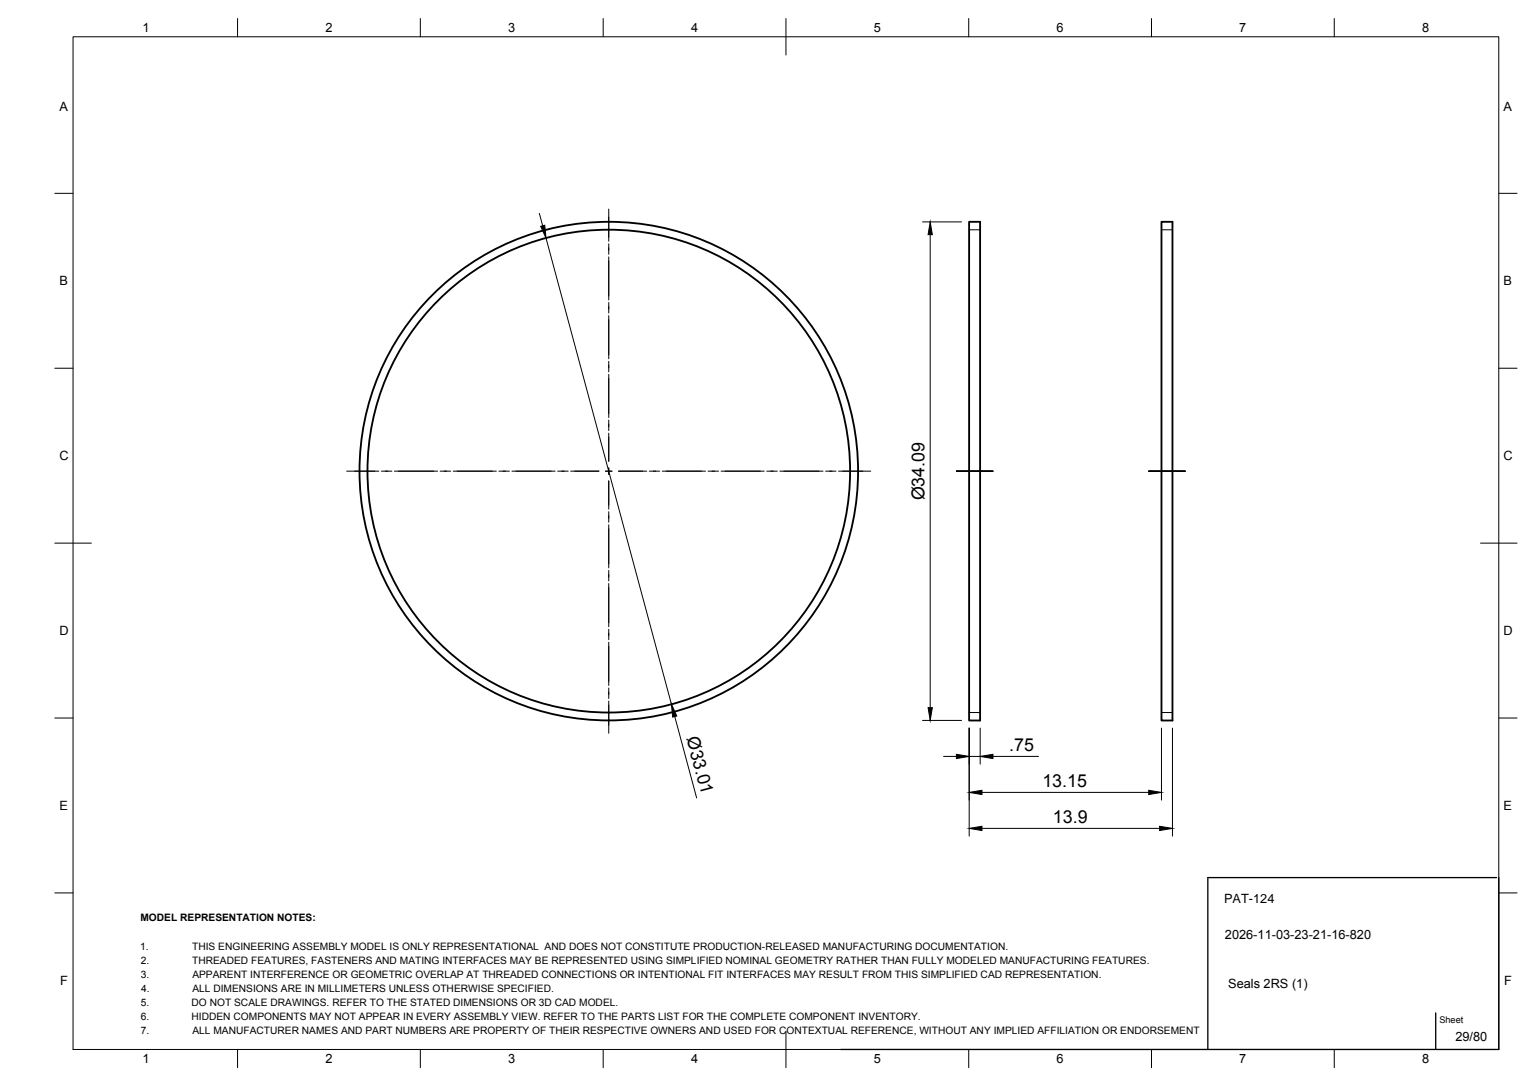
ISO-10303-21;
HEADER;
/* Generated by software containing ST-Developer
 * from STEP Tools, Inc. (www.steptools.com) 
 */

FILE_DESCRIPTION(
/* description */ ('XY cross-slide table'),
/* implementation_level */ '2;1');

FILE_NAME(
/* name */ 'Seals 2RS (1).step',
/* time_stamp */ '2026-10-28T03:22:46-07:00',
/* author */ (''),
/* organization */ (''),
/* preprocessor_version */ 'ST-DEVELOPER v20.2',
/* originating_system */ 'Autodesk Translation Framework v15.17.0.0',
/* authorisation */ '');

FILE_SCHEMA (('AUTOMOTIVE_DESIGN { 1 0 10303 214 3 1 1 }'));
ENDSEC;

DATA;
#10=MECHANICAL_DESIGN_GEOMETRIC_PRESENTATION_REPRESENTATION('',(#1704,#1705),#62984);
#1524=SHAPE_REPRESENTATION_RELATIONSHIP('SRR','None',#63374,#1607);
#1607=ADVANCED_BREP_SHAPE_REPRESENTATION('',(#1817,#1818),#62911);
#1704=STYLED_ITEM('',(#63912),#1817);
#1705=STYLED_ITEM('',(#63912),#1818);
#1817=MANIFOLD_SOLID_BREP('Body1',#22998);
#1818=MANIFOLD_SOLID_BREP('Body2',#22999);
#1997=FACE_BOUND('',#4532,.T.);
#1998=FACE_BOUND('',#4535,.T.);
#1999=FACE_BOUND('',#4538,.T.);
#2000=FACE_BOUND('',#4541,.T.);
#2410=PLANE('',#24526);
#2411=PLANE('',#24531);
#2412=PLANE('',#24534);
#2413=PLANE('',#24539);
#3107=FACE_OUTER_BOUND('',#4531,.T.);
#3108=FACE_OUTER_BOUND('',#4533,.T.);
#3109=FACE_OUTER_BOUND('',#4534,.T.);
#3110=FACE_OUTER_BOUND('',#4536,.T.);
#3111=FACE_OUTER_BOUND('',#4537,.T.);
#3112=FACE_OUTER_BOUND('',#4539,.T.);
#3113=FACE_OUTER_BOUND('',#4540,.T.);
#3114=FACE_OUTER_BOUND('',#4542,.T.);
#4531=EDGE_LOOP('',(#15940));
#4532=EDGE_LOOP('',(#15941));
#4533=EDGE_LOOP('',(#15942,#15943,#15944,#15945));
#4534=EDGE_LOOP('',(#15946));
#4535=EDGE_LOOP('',(#15947));
#4536=EDGE_LOOP('',(#15948,#15949,#15950,#15951));
#4537=EDGE_LOOP('',(#15952));
#4538=EDGE_LOOP('',(#15953));
#4539=EDGE_LOOP('',(#15954,#15955,#15956,#15957));
#4540=EDGE_LOOP('',(#15958));
#4541=EDGE_LOOP('',(#15959));
#4542=EDGE_LOOP('',(#15960,#15961,#15962,#15963));
#6135=LINE('',#34657,#7622);
#6136=LINE('',#34662,#7623);
#6137=LINE('',#34671,#7624);
#6138=LINE('',#34676,#7625);
#7622=VECTOR('',#27752,1.70469);
#7623=VECTOR('',#27759,1.65031);
#7624=VECTOR('',#27770,1.70469);
#7625=VECTOR('',#27777,1.65031);
#9137=CIRCLE('',#24527,1.70469);
#9138=CIRCLE('',#24528,1.65031);
#9139=CIRCLE('',#24530,1.70469);
#9140=CIRCLE('',#24532,1.65031);
#9141=CIRCLE('',#24535,1.70469);
#9142=CIRCLE('',#24536,1.65031);
#9143=CIRCLE('',#24538,1.70469);
#9144=CIRCLE('',#24540,1.65031);
#10133=VERTEX_POINT('',#34650);
#10134=VERTEX_POINT('',#34652);
#10135=VERTEX_POINT('',#34655);
#10136=VERTEX_POINT('',#34659);
#10137=VERTEX_POINT('',#34664);
#10138=VERTEX_POINT('',#34666);
#10139=VERTEX_POINT('',#34669);
#10140=VERTEX_POINT('',#34673);
#12354=EDGE_CURVE('',#10133,#10133,#9137,.T.);
#12355=EDGE_CURVE('',#10134,#10134,#9138,.T.);
#12356=EDGE_CURVE('',#10135,#10135,#9139,.T.);
#12357=EDGE_CURVE('',#10135,#10133,#6135,.T.);
#12358=EDGE_CURVE('',#10136,#10136,#9140,.T.);
#12359=EDGE_CURVE('',#10136,#10134,#6136,.T.);
#12360=EDGE_CURVE('',#10137,#10137,#9141,.T.);
#12361=EDGE_CURVE('',#10138,#10138,#9142,.T.);
#12362=EDGE_CURVE('',#10139,#10139,#9143,.T.);
#12363=EDGE_CURVE('',#10139,#10137,#6137,.T.);
#12364=EDGE_CURVE('',#10140,#10140,#9144,.T.);
#12365=EDGE_CURVE('',#10140,#10138,#6138,.T.);
#15940=ORIENTED_EDGE('',*,*,#12354,.F.);
#15941=ORIENTED_EDGE('',*,*,#12355,.T.);
#15942=ORIENTED_EDGE('',*,*,#12356,.F.);
#15943=ORIENTED_EDGE('',*,*,#12357,.T.);
#15944=ORIENTED_EDGE('',*,*,#12354,.T.);
#15945=ORIENTED_EDGE('',*,*,#12357,.F.);
#15946=ORIENTED_EDGE('',*,*,#12356,.T.);
#15947=ORIENTED_EDGE('',*,*,#12358,.F.);
#15948=ORIENTED_EDGE('',*,*,#12358,.T.);
#15949=ORIENTED_EDGE('',*,*,#12359,.T.);
#15950=ORIENTED_EDGE('',*,*,#12355,.F.);
#15951=ORIENTED_EDGE('',*,*,#12359,.F.);
#15952=ORIENTED_EDGE('',*,*,#12360,.F.);
#15953=ORIENTED_EDGE('',*,*,#12361,.T.);
#15954=ORIENTED_EDGE('',*,*,#12362,.F.);
#15955=ORIENTED_EDGE('',*,*,#12363,.T.);
#15956=ORIENTED_EDGE('',*,*,#12360,.T.);
#15957=ORIENTED_EDGE('',*,*,#12363,.F.);
#15958=ORIENTED_EDGE('',*,*,#12362,.T.);
#15959=ORIENTED_EDGE('',*,*,#12364,.F.);
#15960=ORIENTED_EDGE('',*,*,#12364,.T.);
#15961=ORIENTED_EDGE('',*,*,#12365,.T.);
#15962=ORIENTED_EDGE('',*,*,#12361,.F.);
#15963=ORIENTED_EDGE('',*,*,#12365,.F.);
#21122=CYLINDRICAL_SURFACE('',#24529,1.70469);
#21123=CYLINDRICAL_SURFACE('',#24533,1.65031);
#21124=CYLINDRICAL_SURFACE('',#24537,1.70469);
#21125=CYLINDRICAL_SURFACE('',#24541,1.65031);
#21888=ADVANCED_FACE('',(#3107,#1997),#2410,.T.);
#21889=ADVANCED_FACE('',(#3108),#21122,.T.);
#21890=ADVANCED_FACE('',(#3109,#1998),#2411,.T.);
#21891=ADVANCED_FACE('',(#3110),#21123,.F.);
#21892=ADVANCED_FACE('',(#3111,#1999),#2412,.T.);
#21893=ADVANCED_FACE('',(#3112),#21124,.T.);
#21894=ADVANCED_FACE('',(#3113,#2000),#2413,.T.);
#21895=ADVANCED_FACE('',(#3114),#21125,.F.);
#22998=CLOSED_SHELL('',(#21888,#21889,#21890,#21891));
#22999=CLOSED_SHELL('',(#21892,#21893,#21894,#21895));
#24525=AXIS2_PLACEMENT_3D('',#34648,#27740,#27741);
#24526=AXIS2_PLACEMENT_3D('',#34649,#27742,#27743);
#24527=AXIS2_PLACEMENT_3D('',#34651,#27744,#27745);
#24528=AXIS2_PLACEMENT_3D('',#34653,#27746,#27747);
#24529=AXIS2_PLACEMENT_3D('',#34654,#27748,#27749);
#24530=AXIS2_PLACEMENT_3D('',#34656,#27750,#27751);
#24531=AXIS2_PLACEMENT_3D('',#34658,#27753,#27754);
#24532=AXIS2_PLACEMENT_3D('',#34660,#27755,#27756);
#24533=AXIS2_PLACEMENT_3D('',#34661,#27757,#27758);
#24534=AXIS2_PLACEMENT_3D('',#34663,#27760,#27761);
#24535=AXIS2_PLACEMENT_3D('',#34665,#27762,#27763);
#24536=AXIS2_PLACEMENT_3D('',#34667,#27764,#27765);
#24537=AXIS2_PLACEMENT_3D('',#34668,#27766,#27767);
#24538=AXIS2_PLACEMENT_3D('',#34670,#27768,#27769);
#24539=AXIS2_PLACEMENT_3D('',#34672,#27771,#27772);
#24540=AXIS2_PLACEMENT_3D('',#34674,#27773,#27774);
#24541=AXIS2_PLACEMENT_3D('',#34675,#27775,#27776);
#27740=DIRECTION('axis',(0.,0.,1.));
#27741=DIRECTION('refdir',(1.,0.,0.));
#27742=DIRECTION('center_axis',(0.,1.,0.));
#27743=DIRECTION('ref_axis',(0.,0.,1.));
#27744=DIRECTION('center_axis',(0.,-1.,0.));
#27745=DIRECTION('ref_axis',(1.,0.,0.));
#27746=DIRECTION('center_axis',(0.,-1.,0.));
#27747=DIRECTION('ref_axis',(1.,0.,0.));
#27748=DIRECTION('center_axis',(0.,-1.,0.));
#27749=DIRECTION('ref_axis',(1.,0.,0.));
#27750=DIRECTION('center_axis',(0.,-1.,0.));
#27751=DIRECTION('ref_axis',(1.,0.,0.));
#27752=DIRECTION('',(0.,1.,0.));
#27753=DIRECTION('center_axis',(0.,-1.,0.));
#27754=DIRECTION('ref_axis',(0.,0.,-1.));
#27755=DIRECTION('center_axis',(0.,-1.,0.));
#27756=DIRECTION('ref_axis',(1.,0.,0.));
#27757=DIRECTION('center_axis',(0.,-1.,0.));
#27758=DIRECTION('ref_axis',(1.,0.,0.));
#27759=DIRECTION('',(0.,1.,0.));
#27760=DIRECTION('center_axis',(0.,1.,0.));
#27761=DIRECTION('ref_axis',(0.,0.,1.));
#27762=DIRECTION('center_axis',(0.,-1.,0.));
#27763=DIRECTION('ref_axis',(1.,0.,0.));
#27764=DIRECTION('center_axis',(0.,-1.,0.));
#27765=DIRECTION('ref_axis',(1.,0.,0.));
#27766=DIRECTION('center_axis',(0.,-1.,0.));
#27767=DIRECTION('ref_axis',(1.,0.,0.));
#27768=DIRECTION('center_axis',(0.,-1.,0.));
#27769=DIRECTION('ref_axis',(1.,0.,0.));
#27770=DIRECTION('',(0.,1.,0.));
#27771=DIRECTION('center_axis',(0.,-1.,0.));
#27772=DIRECTION('ref_axis',(0.,0.,-1.));
#27773=DIRECTION('center_axis',(0.,-1.,0.));
#27774=DIRECTION('ref_axis',(1.,0.,0.));
#27775=DIRECTION('center_axis',(0.,-1.,0.));
#27776=DIRECTION('ref_axis',(1.,0.,0.));
#27777=DIRECTION('',(0.,1.,0.));
#34648=CARTESIAN_POINT('',(0.,0.,0.));
#34649=CARTESIAN_POINT('Origin',(1.70469,0.695,0.));
#34650=CARTESIAN_POINT('',(-1.70469,0.695,-2.0876431520385E-16));
#34651=CARTESIAN_POINT('Origin',(0.,0.695,0.));
#34652=CARTESIAN_POINT('',(-1.65031,0.695,-2.02104685910087E-16));
#34653=CARTESIAN_POINT('Origin',(0.,0.695,0.));
#34654=CARTESIAN_POINT('Origin',(0.,0.6575,0.));
#34655=CARTESIAN_POINT('',(-1.70469,0.62,-2.0876431520385E-16));
#34656=CARTESIAN_POINT('Origin',(0.,0.62,0.));
#34657=CARTESIAN_POINT('',(-1.70469,0.6575,-2.0876431520385E-16));
#34658=CARTESIAN_POINT('Origin',(1.65031,0.62,0.));
#34659=CARTESIAN_POINT('',(-1.65031,0.62,-2.02104685910087E-16));
#34660=CARTESIAN_POINT('Origin',(0.,0.62,0.));
#34661=CARTESIAN_POINT('Origin',(0.,0.6575,0.));
#34662=CARTESIAN_POINT('',(-1.65031,0.6575,-2.02104685910087E-16));
#34663=CARTESIAN_POINT('Origin',(1.70469,-0.62,0.));
#34664=CARTESIAN_POINT('',(-1.70469,-0.62,-2.0876431520385E-16));
#34665=CARTESIAN_POINT('Origin',(0.,-0.62,0.));
#34666=CARTESIAN_POINT('',(-1.65031,-0.62,-2.02104685910087E-16));
#34667=CARTESIAN_POINT('Origin',(0.,-0.62,0.));
#34668=CARTESIAN_POINT('Origin',(0.,-0.6575,0.));
#34669=CARTESIAN_POINT('',(-1.70469,-0.695,-2.0876431520385E-16));
#34670=CARTESIAN_POINT('Origin',(0.,-0.695,0.));
#34671=CARTESIAN_POINT('',(-1.70469,-0.6575,-2.0876431520385E-16));
#34672=CARTESIAN_POINT('Origin',(1.65031,-0.695,0.));
#34673=CARTESIAN_POINT('',(-1.65031,-0.695,-2.02104685910087E-16));
#34674=CARTESIAN_POINT('Origin',(0.,-0.695,0.));
#34675=CARTESIAN_POINT('Origin',(0.,-0.6575,0.));
#34676=CARTESIAN_POINT('',(-1.65031,-0.6575,-2.02104685910087E-16));
#62812=UNCERTAINTY_MEASURE_WITH_UNIT(LENGTH_MEASURE(0.001),#62985,
'DISTANCE_ACCURACY_VALUE',
'Maximum model space distance between geometric entities at asserted c
onnectivities');
#62885=UNCERTAINTY_MEASURE_WITH_UNIT(LENGTH_MEASURE(0.001),#62985,
'DISTANCE_ACCURACY_VALUE',
'Maximum model space distance between geometric entities at asserted c
onnectivities');
#62911=(
GEOMETRIC_REPRESENTATION_CONTEXT(3)
GLOBAL_UNCERTAINTY_ASSIGNED_CONTEXT((#62812))
GLOBAL_UNIT_ASSIGNED_CONTEXT((#62985,#62987,#62988))
REPRESENTATION_CONTEXT('','3D')
);
#62984=(
GEOMETRIC_REPRESENTATION_CONTEXT(3)
GLOBAL_UNCERTAINTY_ASSIGNED_CONTEXT((#62885))
GLOBAL_UNIT_ASSIGNED_CONTEXT((#62985,#62987,#62988))
REPRESENTATION_CONTEXT('','3D')
);
#62985=(
LENGTH_UNIT()
NAMED_UNIT(*)
SI_UNIT(.CENTI.,.METRE.)
);
#62987=(
NAMED_UNIT(*)
PLANE_ANGLE_UNIT()
SI_UNIT($,.RADIAN.)
);
#62988=(
NAMED_UNIT(*)
SI_UNIT($,.STERADIAN.)
SOLID_ANGLE_UNIT()
);
#63014=SHAPE_DEFINITION_REPRESENTATION(#63117,#63374);
#63117=PRODUCT_DEFINITION_SHAPE('',$,#63473);
#63374=SHAPE_REPRESENTATION('',(#24525),#62911);
#63447=PRODUCT_DEFINITION_CONTEXT('part definition',#63743,'design');
#63473=PRODUCT_DEFINITION('Seals 2RS (1)','Seals 2RS (1)',#63571,#63447);
#63571=PRODUCT_DEFINITION_FORMATION('',$,#63770);
#63743=APPLICATION_CONTEXT(
'Core Data for Automotive Mechanical Design Process');
#63744=PRODUCT_CONTEXT('part definition',#63743,'mechanical');
#63770=PRODUCT('Seals 2RS (1)','Seals 2RS (1)','Seals 2RS (1)',(#63744));
#63906=COLOUR_RGB('Grey',0.48,0.52,0.57);
#63907=FILL_AREA_STYLE_COLOUR('',#63906);
#63908=FILL_AREA_STYLE('',(#63907));
#63909=SURFACE_STYLE_FILL_AREA(#63908);
#63910=SURFACE_SIDE_STYLE('',(#63909));
#63911=SURFACE_STYLE_USAGE(.BOTH.,#63910);
#63912=PRESENTATION_STYLE_ASSIGNMENT((#63911));
ENDSEC;
END-ISO-10303-21;
